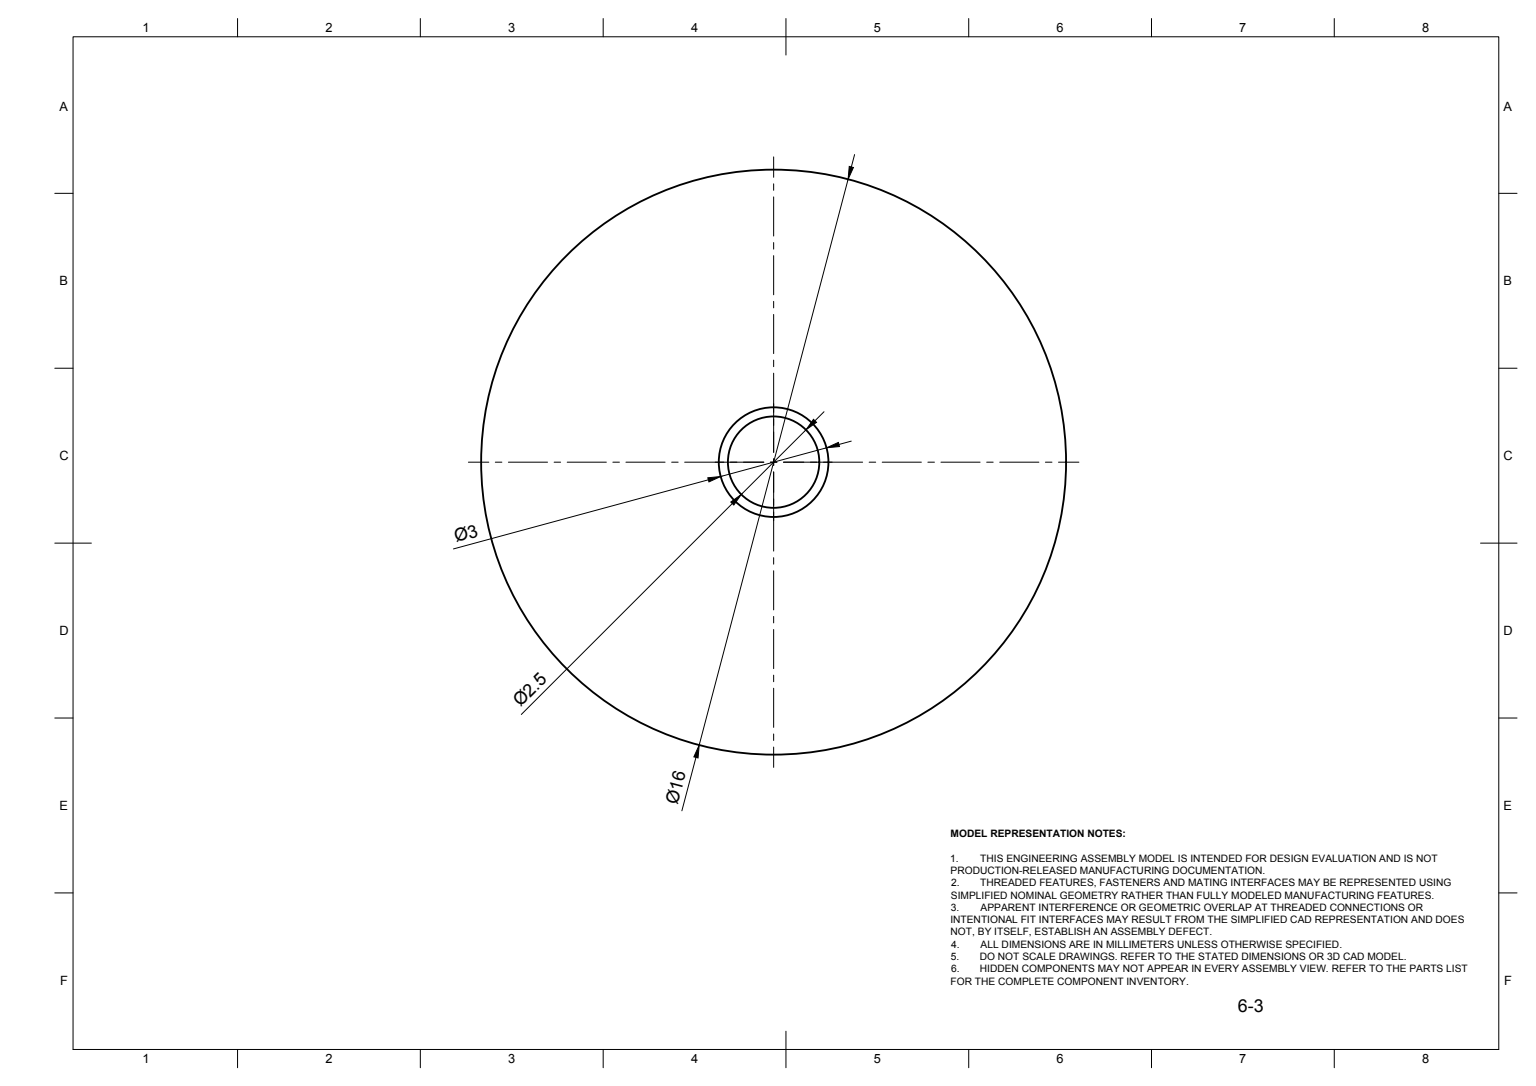
ISO-10303-21;
HEADER;
/* Generated by software containing ST-Developer
 * from STEP Tools, Inc. (www.steptools.com) 
 */

FILE_DESCRIPTION(
/* description */ (''),
/* implementation_level */ '2;1');

FILE_NAME(
/* name */ '6-3.step',
/* time_stamp */ '2026-10-06T01:16:10-07:00',
/* author */ (''),
/* organization */ (''),
/* preprocessor_version */ 'ST-DEVELOPER v20.2',
/* originating_system */ 'Autodesk Translation Framework v15.15.0.0',
/* authorisation */ '');

FILE_SCHEMA (('AUTOMOTIVE_DESIGN { 1 0 10303 214 3 1 1 }'));
ENDSEC;

DATA;
#10=MECHANICAL_DESIGN_GEOMETRIC_PRESENTATION_REPRESENTATION('',(#327,#328),#17113);
#238=OPEN_SHELL('',(#5993,#5994));
#256=SHELL_BASED_SURFACE_MODEL('Body2',(#238));
#278=SHAPE_REPRESENTATION_RELATIONSHIP('SRR','None',#17204,#294);
#294=ADVANCED_BREP_SHAPE_REPRESENTATION('',(#344),#17111);
#327=STYLED_ITEM('',(#17298),#344);
#328=STYLED_ITEM('',(#17298),#256);
#344=MANIFOLD_SOLID_BREP('Body1',#6030);
#489=CYLINDRICAL_SURFACE('',#6905,1.25);
#490=CYLINDRICAL_SURFACE('',#6909,8.);
#491=CYLINDRICAL_SURFACE('',#6913,6.75);
#492=CYLINDRICAL_SURFACE('',#6917,8.);
#493=CYLINDRICAL_SURFACE('',#6918,1.5);
#626=FACE_BOUND('',#1820,.T.);
#627=FACE_BOUND('',#1823,.T.);
#628=FACE_BOUND('',#1826,.T.);
#629=FACE_BOUND('',#1829,.T.);
#630=FACE_BOUND('',#1833,.T.);
#977=CIRCLE('',#6903,8.);
#978=CIRCLE('',#6904,1.25);
#979=CIRCLE('',#6906,1.25);
#980=CIRCLE('',#6908,8.);
#981=CIRCLE('',#6910,8.);
#982=CIRCLE('',#6912,6.75);
#983=CIRCLE('',#6914,6.75);
#984=CIRCLE('',#6916,8.);
#985=CIRCLE('',#6919,1.5);
#986=CIRCLE('',#6920,1.5);
#987=CIRCLE('',#6922,1.25);
#1337=FACE_OUTER_BOUND('',#1819,.T.);
#1338=FACE_OUTER_BOUND('',#1821,.T.);
#1339=FACE_OUTER_BOUND('',#1822,.T.);
#1340=FACE_OUTER_BOUND('',#1824,.T.);
#1341=FACE_OUTER_BOUND('',#1825,.T.);
#1342=FACE_OUTER_BOUND('',#1827,.T.);
#1343=FACE_OUTER_BOUND('',#1828,.T.);
#1344=FACE_OUTER_BOUND('',#1830,.T.);
#1345=FACE_OUTER_BOUND('',#1831,.T.);
#1346=FACE_OUTER_BOUND('',#1832,.T.);
#1819=EDGE_LOOP('',(#5366));
#1820=EDGE_LOOP('',(#5367));
#1821=EDGE_LOOP('',(#5368,#5369,#5370,#5371));
#1822=EDGE_LOOP('',(#5372));
#1823=EDGE_LOOP('',(#5373));
#1824=EDGE_LOOP('',(#5374,#5375,#5376,#5377));
#1825=EDGE_LOOP('',(#5378));
#1826=EDGE_LOOP('',(#5379));
#1827=EDGE_LOOP('',(#5380,#5381,#5382,#5383));
#1828=EDGE_LOOP('',(#5384));
#1829=EDGE_LOOP('',(#5385));
#1830=EDGE_LOOP('',(#5386,#5387,#5388,#5389));
#1831=EDGE_LOOP('',(#5390,#5391,#5392,#5393));
#1832=EDGE_LOOP('',(#5394));
#1833=EDGE_LOOP('',(#5395));
#2182=LINE('',#16913,#2543);
#2183=LINE('',#16920,#2544);
#2184=LINE('',#16927,#2545);
#2185=LINE('',#16933,#2546);
#2186=LINE('',#16938,#2547);
#2543=VECTOR('',#8694,1.25);
#2544=VECTOR('',#8703,8.);
#2545=VECTOR('',#8712,6.75);
#2546=VECTOR('',#8721,8.);
#2547=VECTOR('',#8726,1.5);
#3057=VERTEX_POINT('',#16907);
#3058=VERTEX_POINT('',#16909);
#3059=VERTEX_POINT('',#16912);
#3060=VERTEX_POINT('',#16916);
#3061=VERTEX_POINT('',#16919);
#3062=VERTEX_POINT('',#16923);
#3063=VERTEX_POINT('',#16926);
#3064=VERTEX_POINT('',#16930);
#3065=VERTEX_POINT('',#16935);
#3066=VERTEX_POINT('',#16937);
#3067=VERTEX_POINT('',#16941);
#3846=EDGE_CURVE('',#3057,#3057,#977,.T.);
#3847=EDGE_CURVE('',#3058,#3058,#978,.T.);
#3848=EDGE_CURVE('',#3058,#3059,#2182,.T.);
#3849=EDGE_CURVE('',#3059,#3059,#979,.T.);
#3850=EDGE_CURVE('',#3060,#3060,#980,.T.);
#3851=EDGE_CURVE('',#3060,#3061,#2183,.T.);
#3852=EDGE_CURVE('',#3061,#3061,#981,.T.);
#3853=EDGE_CURVE('',#3062,#3062,#982,.T.);
#3854=EDGE_CURVE('',#3062,#3063,#2184,.T.);
#3855=EDGE_CURVE('',#3063,#3063,#983,.T.);
#3856=EDGE_CURVE('',#3064,#3064,#984,.T.);
#3857=EDGE_CURVE('',#3064,#3057,#2185,.T.);
#3858=EDGE_CURVE('',#3065,#3065,#985,.T.);
#3859=EDGE_CURVE('',#3065,#3066,#2186,.T.);
#3860=EDGE_CURVE('',#3066,#3066,#986,.T.);
#3861=EDGE_CURVE('',#3067,#3067,#987,.T.);
#5366=ORIENTED_EDGE('',*,*,#3846,.T.);
#5367=ORIENTED_EDGE('',*,*,#3847,.T.);
#5368=ORIENTED_EDGE('',*,*,#3847,.F.);
#5369=ORIENTED_EDGE('',*,*,#3848,.T.);
#5370=ORIENTED_EDGE('',*,*,#3849,.T.);
#5371=ORIENTED_EDGE('',*,*,#3848,.F.);
#5372=ORIENTED_EDGE('',*,*,#3850,.T.);
#5373=ORIENTED_EDGE('',*,*,#3849,.F.);
#5374=ORIENTED_EDGE('',*,*,#3850,.F.);
#5375=ORIENTED_EDGE('',*,*,#3851,.T.);
#5376=ORIENTED_EDGE('',*,*,#3852,.T.);
#5377=ORIENTED_EDGE('',*,*,#3851,.F.);
#5378=ORIENTED_EDGE('',*,*,#3852,.F.);
#5379=ORIENTED_EDGE('',*,*,#3853,.T.);
#5380=ORIENTED_EDGE('',*,*,#3853,.F.);
#5381=ORIENTED_EDGE('',*,*,#3854,.T.);
#5382=ORIENTED_EDGE('',*,*,#3855,.T.);
#5383=ORIENTED_EDGE('',*,*,#3854,.F.);
#5384=ORIENTED_EDGE('',*,*,#3856,.T.);
#5385=ORIENTED_EDGE('',*,*,#3855,.F.);
#5386=ORIENTED_EDGE('',*,*,#3856,.F.);
#5387=ORIENTED_EDGE('',*,*,#3857,.T.);
#5388=ORIENTED_EDGE('',*,*,#3846,.F.);
#5389=ORIENTED_EDGE('',*,*,#3857,.F.);
#5390=ORIENTED_EDGE('',*,*,#3858,.F.);
#5391=ORIENTED_EDGE('',*,*,#3859,.T.);
#5392=ORIENTED_EDGE('',*,*,#3860,.T.);
#5393=ORIENTED_EDGE('',*,*,#3859,.F.);
#5394=ORIENTED_EDGE('',*,*,#3860,.F.);
#5395=ORIENTED_EDGE('',*,*,#3861,.F.);
#5640=PLANE('',#6902);
#5641=PLANE('',#6907);
#5642=PLANE('',#6911);
#5643=PLANE('',#6915);
#5644=PLANE('',#6921);
#5985=ADVANCED_FACE('',(#1337,#626),#5640,.F.);
#5986=ADVANCED_FACE('',(#1338),#489,.F.);
#5987=ADVANCED_FACE('',(#1339,#627),#5641,.T.);
#5988=ADVANCED_FACE('',(#1340),#490,.T.);
#5989=ADVANCED_FACE('',(#1341,#628),#5642,.F.);
#5990=ADVANCED_FACE('',(#1342),#491,.T.);
#5991=ADVANCED_FACE('',(#1343,#629),#5643,.T.);
#5992=ADVANCED_FACE('',(#1344),#492,.T.);
#5993=ADVANCED_FACE('',(#1345),#493,.T.);
#5994=ADVANCED_FACE('',(#1346,#630),#5644,.F.);
#6030=CLOSED_SHELL('',(#5985,#5986,#5987,#5988,#5989,#5990,#5991,#5992));
#6901=AXIS2_PLACEMENT_3D('',#16905,#8684,#8685);
#6902=AXIS2_PLACEMENT_3D('',#16906,#8686,#8687);
#6903=AXIS2_PLACEMENT_3D('',#16908,#8688,#8689);
#6904=AXIS2_PLACEMENT_3D('',#16910,#8690,#8691);
#6905=AXIS2_PLACEMENT_3D('',#16911,#8692,#8693);
#6906=AXIS2_PLACEMENT_3D('',#16914,#8695,#8696);
#6907=AXIS2_PLACEMENT_3D('',#16915,#8697,#8698);
#6908=AXIS2_PLACEMENT_3D('',#16917,#8699,#8700);
#6909=AXIS2_PLACEMENT_3D('',#16918,#8701,#8702);
#6910=AXIS2_PLACEMENT_3D('',#16921,#8704,#8705);
#6911=AXIS2_PLACEMENT_3D('',#16922,#8706,#8707);
#6912=AXIS2_PLACEMENT_3D('',#16924,#8708,#8709);
#6913=AXIS2_PLACEMENT_3D('',#16925,#8710,#8711);
#6914=AXIS2_PLACEMENT_3D('',#16928,#8713,#8714);
#6915=AXIS2_PLACEMENT_3D('',#16929,#8715,#8716);
#6916=AXIS2_PLACEMENT_3D('',#16931,#8717,#8718);
#6917=AXIS2_PLACEMENT_3D('',#16932,#8719,#8720);
#6918=AXIS2_PLACEMENT_3D('',#16934,#8722,#8723);
#6919=AXIS2_PLACEMENT_3D('',#16936,#8724,#8725);
#6920=AXIS2_PLACEMENT_3D('',#16939,#8727,#8728);
#6921=AXIS2_PLACEMENT_3D('',#16940,#8729,#8730);
#6922=AXIS2_PLACEMENT_3D('',#16942,#8731,#8732);
#8684=DIRECTION('axis',(0.,0.,1.));
#8685=DIRECTION('refdir',(1.,0.,0.));
#8686=DIRECTION('center_axis',(0.,0.,-1.));
#8687=DIRECTION('ref_axis',(0.,-1.,0.));
#8688=DIRECTION('center_axis',(0.,0.,1.));
#8689=DIRECTION('ref_axis',(0.,-1.,0.));
#8690=DIRECTION('center_axis',(0.,0.,-1.));
#8691=DIRECTION('ref_axis',(0.,-1.,0.));
#8692=DIRECTION('center_axis',(0.,0.,-1.));
#8693=DIRECTION('ref_axis',(0.,-1.,0.));
#8694=DIRECTION('',(0.,0.,-1.));
#8695=DIRECTION('center_axis',(0.,0.,-1.));
#8696=DIRECTION('ref_axis',(0.,-1.,0.));
#8697=DIRECTION('center_axis',(0.,0.,-1.));
#8698=DIRECTION('ref_axis',(0.,-1.,0.));
#8699=DIRECTION('center_axis',(0.,0.,-1.));
#8700=DIRECTION('ref_axis',(0.,-1.,0.));
#8701=DIRECTION('center_axis',(0.,0.,-1.));
#8702=DIRECTION('ref_axis',(0.,-1.,0.));
#8703=DIRECTION('',(0.,0.,1.));
#8704=DIRECTION('center_axis',(0.,0.,-1.));
#8705=DIRECTION('ref_axis',(0.,-1.,0.));
#8706=DIRECTION('center_axis',(0.,0.,-1.));
#8707=DIRECTION('ref_axis',(0.,-1.,0.));
#8708=DIRECTION('center_axis',(0.,0.,-1.));
#8709=DIRECTION('ref_axis',(0.,-1.,0.));
#8710=DIRECTION('center_axis',(0.,0.,-1.));
#8711=DIRECTION('ref_axis',(0.,-1.,0.));
#8712=DIRECTION('',(0.,0.,1.));
#8713=DIRECTION('center_axis',(0.,0.,-1.));
#8714=DIRECTION('ref_axis',(0.,-1.,0.));
#8715=DIRECTION('center_axis',(0.,0.,-1.));
#8716=DIRECTION('ref_axis',(0.,-1.,0.));
#8717=DIRECTION('center_axis',(0.,0.,-1.));
#8718=DIRECTION('ref_axis',(0.,-1.,0.));
#8719=DIRECTION('center_axis',(0.,0.,-1.));
#8720=DIRECTION('ref_axis',(0.,-1.,0.));
#8721=DIRECTION('',(0.,0.,1.));
#8722=DIRECTION('center_axis',(0.,0.,-1.));
#8723=DIRECTION('ref_axis',(-1.,0.,0.));
#8724=DIRECTION('center_axis',(0.,0.,-1.));
#8725=DIRECTION('ref_axis',(1.,0.,0.));
#8726=DIRECTION('',(0.,0.,1.));
#8727=DIRECTION('center_axis',(0.,0.,-1.));
#8728=DIRECTION('ref_axis',(1.,0.,0.));
#8729=DIRECTION('center_axis',(0.,0.,-1.));
#8730=DIRECTION('ref_axis',(-1.,0.,0.));
#8731=DIRECTION('center_axis',(0.,0.,1.));
#8732=DIRECTION('ref_axis',(1.,0.,0.));
#16905=CARTESIAN_POINT('',(0.,0.,0.));
#16906=CARTESIAN_POINT('Origin',(0.,0.,0.));
#16907=CARTESIAN_POINT('',(0.,8.,0.));
#16908=CARTESIAN_POINT('Origin',(0.,0.,0.));
#16909=CARTESIAN_POINT('',(0.,1.25,0.));
#16910=CARTESIAN_POINT('Origin',(0.,0.,0.));
#16911=CARTESIAN_POINT('Origin',(0.,0.,0.4));
#16912=CARTESIAN_POINT('',(0.,1.25,-8.));
#16913=CARTESIAN_POINT('',(1.53080849893419E-16,1.25,0.4));
#16914=CARTESIAN_POINT('Origin',(0.,0.,-8.));
#16915=CARTESIAN_POINT('Origin',(0.,0.,-8.));
#16916=CARTESIAN_POINT('',(0.,8.,-8.));
#16917=CARTESIAN_POINT('Origin',(0.,0.,-8.));
#16918=CARTESIAN_POINT('Origin',(0.,0.,0.4));
#16919=CARTESIAN_POINT('',(0.,8.,-4.75));
#16920=CARTESIAN_POINT('',(9.79717439317883E-16,8.,0.4));
#16921=CARTESIAN_POINT('Origin',(0.,0.,-4.75));
#16922=CARTESIAN_POINT('Origin',(0.,0.,-4.75));
#16923=CARTESIAN_POINT('',(0.,6.75,-4.75));
#16924=CARTESIAN_POINT('Origin',(0.,0.,-4.75));
#16925=CARTESIAN_POINT('Origin',(0.,0.,0.4));
#16926=CARTESIAN_POINT('',(0.,6.75,-3.25));
#16927=CARTESIAN_POINT('',(8.26636589424463E-16,6.75,0.4));
#16928=CARTESIAN_POINT('Origin',(0.,0.,-3.25));
#16929=CARTESIAN_POINT('Origin',(0.,0.,-3.25));
#16930=CARTESIAN_POINT('',(0.,8.,-3.25));
#16931=CARTESIAN_POINT('Origin',(0.,0.,-3.25));
#16932=CARTESIAN_POINT('Origin',(0.,0.,0.4));
#16933=CARTESIAN_POINT('',(9.79717439317883E-16,8.,0.4));
#16934=CARTESIAN_POINT('Origin',(0.,0.,-8.));
#16935=CARTESIAN_POINT('',(1.5,-1.83697019872103E-16,-8.));
#16936=CARTESIAN_POINT('Origin',(0.,0.,-8.));
#16937=CARTESIAN_POINT('',(1.5,-1.83697019872103E-16,0.));
#16938=CARTESIAN_POINT('',(1.5,-1.83697019872103E-16,-8.));
#16939=CARTESIAN_POINT('Origin',(0.,0.,0.));
#16940=CARTESIAN_POINT('Origin',(0.,0.,0.));
#16941=CARTESIAN_POINT('',(-1.25,0.,0.));
#16942=CARTESIAN_POINT('Origin',(0.,0.,0.));
#17088=UNCERTAINTY_MEASURE_WITH_UNIT(LENGTH_MEASURE(0.01),#17114,
'DISTANCE_ACCURACY_VALUE',
'Maximum model space distance between geometric entities at asserted c
onnectivities');
#17090=UNCERTAINTY_MEASURE_WITH_UNIT(LENGTH_MEASURE(0.01),#17114,
'DISTANCE_ACCURACY_VALUE',
'Maximum model space distance between geometric entities at asserted c
onnectivities');
#17111=(
GEOMETRIC_REPRESENTATION_CONTEXT(3)
GLOBAL_UNCERTAINTY_ASSIGNED_CONTEXT((#17088))
GLOBAL_UNIT_ASSIGNED_CONTEXT((#17114,#17116,#17117))
REPRESENTATION_CONTEXT('','3D')
);
#17113=(
GEOMETRIC_REPRESENTATION_CONTEXT(3)
GLOBAL_UNCERTAINTY_ASSIGNED_CONTEXT((#17090))
GLOBAL_UNIT_ASSIGNED_CONTEXT((#17114,#17116,#17117))
REPRESENTATION_CONTEXT('','3D')
);
#17114=(
LENGTH_UNIT()
NAMED_UNIT(*)
SI_UNIT(.MILLI.,.METRE.)
);
#17116=(
NAMED_UNIT(*)
PLANE_ANGLE_UNIT()
SI_UNIT($,.RADIAN.)
);
#17117=(
NAMED_UNIT(*)
SI_UNIT($,.STERADIAN.)
SOLID_ANGLE_UNIT()
);
#17138=SHAPE_DEFINITION_REPRESENTATION(#17169,#17204);
#17169=PRODUCT_DEFINITION_SHAPE('',$,#17227);
#17204=SHAPE_REPRESENTATION('',(#6901,#256),#17111);
#17206=PRODUCT_DEFINITION_CONTEXT('part definition',#17274,'design');
#17227=PRODUCT_DEFINITION('6-3','6-3',#17249,#17206);
#17249=PRODUCT_DEFINITION_FORMATION('',$,#17296);
#17274=APPLICATION_CONTEXT(
'Core Data for Automotive Mechanical Design Process');
#17275=PRODUCT_CONTEXT('part definition',#17274,'mechanical');
#17296=PRODUCT('6-3','6-3','NOT SPECIFIED',(#17275));
#17298=PRESENTATION_STYLE_ASSIGNMENT((#17299));
#17299=SURFACE_STYLE_USAGE(.BOTH.,#17300);
#17300=SURFACE_SIDE_STYLE('',(#17301));
#17301=SURFACE_STYLE_FILL_AREA(#17302);
#17302=FILL_AREA_STYLE('Steel - Satin',(#17303));
#17303=FILL_AREA_STYLE_COLOUR('Steel - Satin',#17304);
#17304=COLOUR_RGB('Steel - Satin', 0.09019608, 0.27058824, 0.51372549);
ENDSEC;
END-ISO-10303-21;
